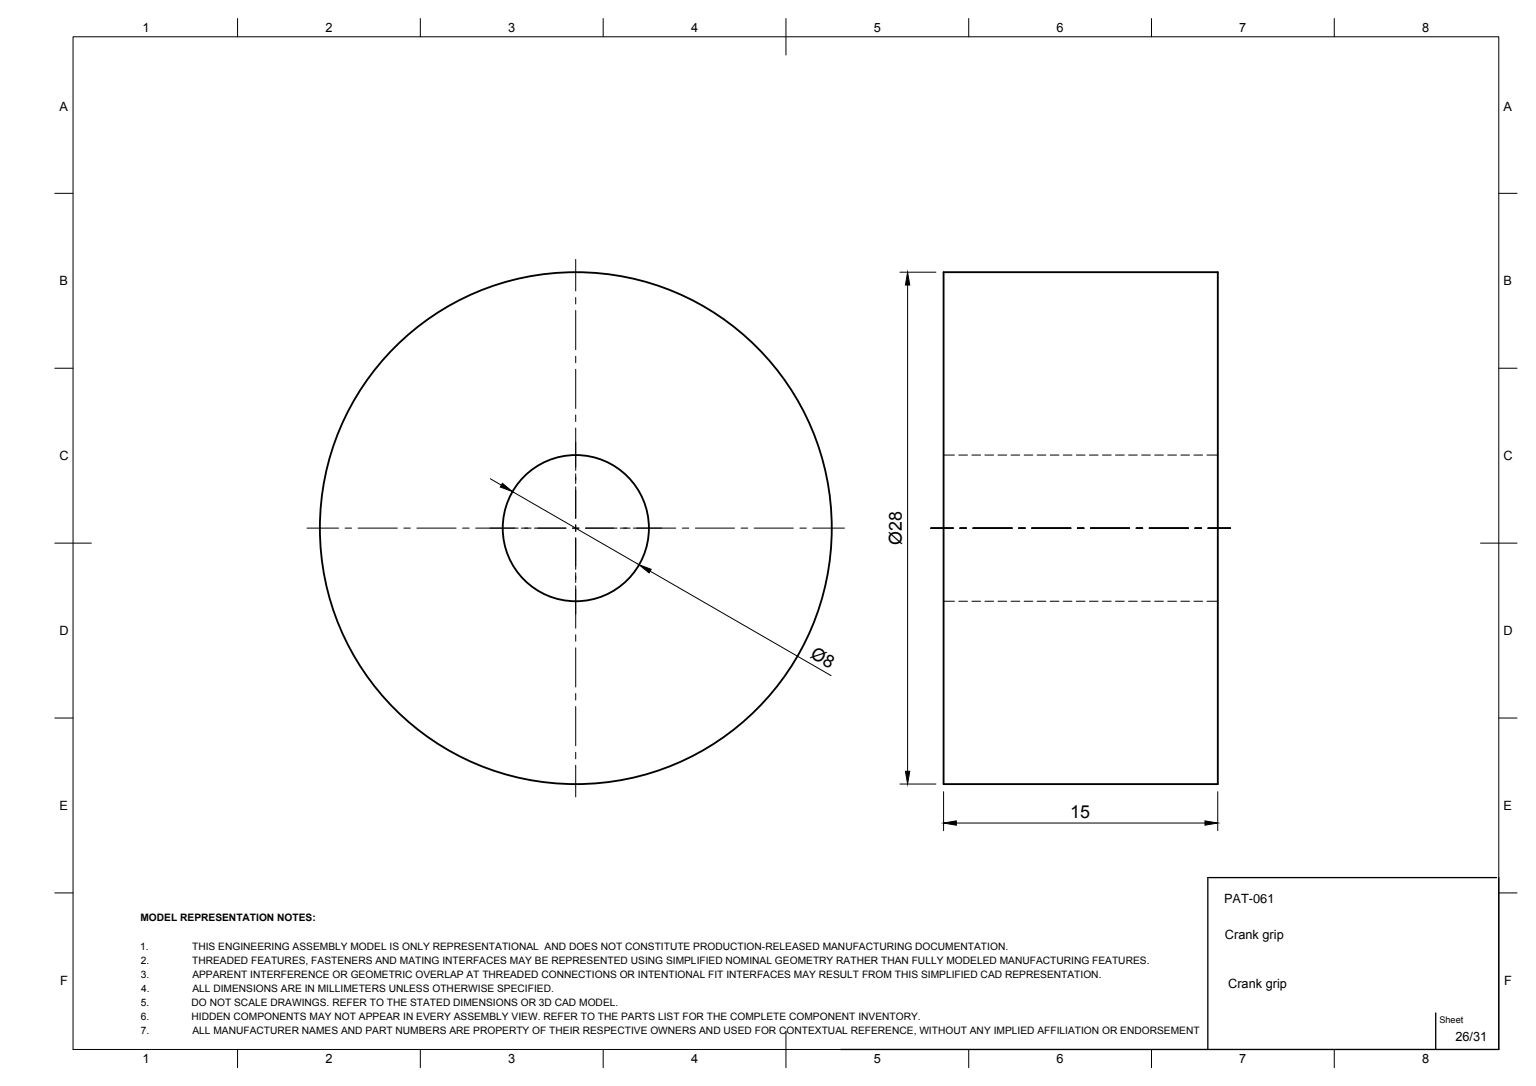
ISO-10303-21;
HEADER;
/* Generated by software containing ST-Developer
 * from STEP Tools, Inc. (www.steptools.com) 
 */

FILE_DESCRIPTION(
/* description */ ('Compact intermittent indexer'),
/* implementation_level */ '2;1');

FILE_NAME(
/* name */ 'Crank grip.step',
/* time_stamp */ '2026-10-29T16:32:17-07:00',
/* author */ (''),
/* organization */ (''),
/* preprocessor_version */ 'ST-DEVELOPER v20.2',
/* originating_system */ 'Autodesk Translation Framework v15.17.0.0',
/* authorisation */ '');

FILE_SCHEMA (('AUTOMOTIVE_DESIGN { 1 0 10303 214 3 1 1 }'));
ENDSEC;

DATA;
#10=MECHANICAL_DESIGN_GEOMETRIC_PRESENTATION_REPRESENTATION('',(#283),#10837);
#227=SHAPE_REPRESENTATION_RELATIONSHIP('SRR','None',#10963,#251);
#251=ADVANCED_BREP_SHAPE_REPRESENTATION('',(#314),#10830);
#283=STYLED_ITEM('',(#11173),#314);
#314=MANIFOLD_SOLID_BREP('Body1',#5656);
#452=FACE_BOUND('',#1314,.T.);
#453=FACE_BOUND('',#1316,.T.);
#587=PLANE('',#6441);
#588=PLANE('',#6442);
#884=FACE_OUTER_BOUND('',#1311,.T.);
#885=FACE_OUTER_BOUND('',#1312,.T.);
#886=FACE_OUTER_BOUND('',#1313,.T.);
#887=FACE_OUTER_BOUND('',#1315,.T.);
#1311=EDGE_LOOP('',(#4660,#4661,#4662,#4663));
#1312=EDGE_LOOP('',(#4664,#4665,#4666,#4667));
#1313=EDGE_LOOP('',(#4668));
#1314=EDGE_LOOP('',(#4669));
#1315=EDGE_LOOP('',(#4670));
#1316=EDGE_LOOP('',(#4671));
#1631=LINE('',#10091,#1989);
#1632=LINE('',#10097,#1990);
#1989=VECTOR('',#7883,0.4);
#1990=VECTOR('',#7890,1.4);
#2395=CIRCLE('',#6436,0.4);
#2396=CIRCLE('',#6437,0.4);
#2397=CIRCLE('',#6439,1.4);
#2398=CIRCLE('',#6440,1.4);
#2807=VERTEX_POINT('',#10088);
#2808=VERTEX_POINT('',#10090);
#2809=VERTEX_POINT('',#10094);
#2810=VERTEX_POINT('',#10096);
#3452=EDGE_CURVE('',#2807,#2807,#2395,.T.);
#3453=EDGE_CURVE('',#2807,#2808,#1631,.T.);
#3454=EDGE_CURVE('',#2808,#2808,#2396,.T.);
#3455=EDGE_CURVE('',#2809,#2809,#2397,.T.);
#3456=EDGE_CURVE('',#2809,#2810,#1632,.T.);
#3457=EDGE_CURVE('',#2810,#2810,#2398,.T.);
#4660=ORIENTED_EDGE('',*,*,#3452,.F.);
#4661=ORIENTED_EDGE('',*,*,#3453,.T.);
#4662=ORIENTED_EDGE('',*,*,#3454,.T.);
#4663=ORIENTED_EDGE('',*,*,#3453,.F.);
#4664=ORIENTED_EDGE('',*,*,#3455,.F.);
#4665=ORIENTED_EDGE('',*,*,#3456,.T.);
#4666=ORIENTED_EDGE('',*,*,#3457,.T.);
#4667=ORIENTED_EDGE('',*,*,#3456,.F.);
#4668=ORIENTED_EDGE('',*,*,#3455,.T.);
#4669=ORIENTED_EDGE('',*,*,#3452,.T.);
#4670=ORIENTED_EDGE('',*,*,#3457,.F.);
#4671=ORIENTED_EDGE('',*,*,#3454,.F.);
#5262=CYLINDRICAL_SURFACE('',#6435,0.4);
#5263=CYLINDRICAL_SURFACE('',#6438,1.4);
#5527=ADVANCED_FACE('',(#884),#5262,.F.);
#5528=ADVANCED_FACE('',(#885),#5263,.T.);
#5529=ADVANCED_FACE('',(#886,#452),#587,.T.);
#5530=ADVANCED_FACE('',(#887,#453),#588,.F.);
#5656=CLOSED_SHELL('',(#5527,#5528,#5529,#5530));
#6434=AXIS2_PLACEMENT_3D('',#10086,#7877,#7878);
#6435=AXIS2_PLACEMENT_3D('',#10087,#7879,#7880);
#6436=AXIS2_PLACEMENT_3D('',#10089,#7881,#7882);
#6437=AXIS2_PLACEMENT_3D('',#10092,#7884,#7885);
#6438=AXIS2_PLACEMENT_3D('',#10093,#7886,#7887);
#6439=AXIS2_PLACEMENT_3D('',#10095,#7888,#7889);
#6440=AXIS2_PLACEMENT_3D('',#10098,#7891,#7892);
#6441=AXIS2_PLACEMENT_3D('',#10099,#7893,#7894);
#6442=AXIS2_PLACEMENT_3D('',#10100,#7895,#7896);
#7877=DIRECTION('axis',(0.,0.,1.));
#7878=DIRECTION('refdir',(1.,0.,0.));
#7879=DIRECTION('center_axis',(0.,0.,1.));
#7880=DIRECTION('ref_axis',(1.,0.,0.));
#7881=DIRECTION('center_axis',(0.,0.,-1.));
#7882=DIRECTION('ref_axis',(1.,0.,0.));
#7883=DIRECTION('',(0.,0.,-1.));
#7884=DIRECTION('center_axis',(0.,0.,-1.));
#7885=DIRECTION('ref_axis',(1.,0.,0.));
#7886=DIRECTION('center_axis',(0.,0.,1.));
#7887=DIRECTION('ref_axis',(1.,0.,0.));
#7888=DIRECTION('center_axis',(0.,0.,1.));
#7889=DIRECTION('ref_axis',(1.,0.,0.));
#7890=DIRECTION('',(0.,0.,-1.));
#7891=DIRECTION('center_axis',(0.,0.,1.));
#7892=DIRECTION('ref_axis',(1.,0.,0.));
#7893=DIRECTION('center_axis',(0.,0.,1.));
#7894=DIRECTION('ref_axis',(1.,0.,0.));
#7895=DIRECTION('center_axis',(0.,0.,1.));
#7896=DIRECTION('ref_axis',(1.,0.,0.));
#10086=CARTESIAN_POINT('',(0.,0.,0.));
#10087=CARTESIAN_POINT('Origin',(0.,0.,7.));
#10088=CARTESIAN_POINT('',(-0.4,-4.89858719658941E-17,8.5));
#10089=CARTESIAN_POINT('Origin',(0.,0.,8.5));
#10090=CARTESIAN_POINT('',(-0.4,-4.89858719658941E-17,7.));
#10091=CARTESIAN_POINT('',(-0.4,-4.89858719658941E-17,7.));
#10092=CARTESIAN_POINT('Origin',(0.,0.,7.));
#10093=CARTESIAN_POINT('Origin',(0.,0.,7.));
#10094=CARTESIAN_POINT('',(-1.4,-1.71450551880629E-16,8.5));
#10095=CARTESIAN_POINT('Origin',(0.,0.,8.5));
#10096=CARTESIAN_POINT('',(-1.4,-1.71450551880629E-16,7.));
#10097=CARTESIAN_POINT('',(-1.4,-1.71450551880629E-16,7.));
#10098=CARTESIAN_POINT('Origin',(0.,0.,7.));
#10099=CARTESIAN_POINT('Origin',(0.,0.,8.5));
#10100=CARTESIAN_POINT('Origin',(0.,0.,7.));
#10800=UNCERTAINTY_MEASURE_WITH_UNIT(LENGTH_MEASURE(0.001),#10838,
'DISTANCE_ACCURACY_VALUE',
'Maximum model space distance between geometric entities at asserted c
onnectivities');
#10807=UNCERTAINTY_MEASURE_WITH_UNIT(LENGTH_MEASURE(0.001),#10838,
'DISTANCE_ACCURACY_VALUE',
'Maximum model space distance between geometric entities at asserted c
onnectivities');
#10830=(
GEOMETRIC_REPRESENTATION_CONTEXT(3)
GLOBAL_UNCERTAINTY_ASSIGNED_CONTEXT((#10800))
GLOBAL_UNIT_ASSIGNED_CONTEXT((#10838,#10840,#10841))
REPRESENTATION_CONTEXT('','3D')
);
#10837=(
GEOMETRIC_REPRESENTATION_CONTEXT(3)
GLOBAL_UNCERTAINTY_ASSIGNED_CONTEXT((#10807))
GLOBAL_UNIT_ASSIGNED_CONTEXT((#10838,#10840,#10841))
REPRESENTATION_CONTEXT('','3D')
);
#10838=(
LENGTH_UNIT()
NAMED_UNIT(*)
SI_UNIT(.CENTI.,.METRE.)
);
#10840=(
NAMED_UNIT(*)
PLANE_ANGLE_UNIT()
SI_UNIT($,.RADIAN.)
);
#10841=(
NAMED_UNIT(*)
SI_UNIT($,.STERADIAN.)
SOLID_ANGLE_UNIT()
);
#10864=SHAPE_DEFINITION_REPRESENTATION(#10898,#10963);
#10898=PRODUCT_DEFINITION_SHAPE('',$,#10993);
#10963=SHAPE_REPRESENTATION('',(#6434),#10830);
#10970=PRODUCT_DEFINITION_CONTEXT('part definition',#11059,'design');
#10993=PRODUCT_DEFINITION('Crank grip','Crank grip',#11022,#10970);
#11022=PRODUCT_DEFINITION_FORMATION('',$,#11083);
#11059=APPLICATION_CONTEXT(
'Core Data for Automotive Mechanical Design Process');
#11060=PRODUCT_CONTEXT('part definition',#11059,'mechanical');
#11083=PRODUCT('Crank grip','Crank grip','Crank grip',(#11060));
#11167=COLOUR_RGB('Black',0.12,0.14,0.17);
#11168=FILL_AREA_STYLE_COLOUR('',#11167);
#11169=FILL_AREA_STYLE('',(#11168));
#11170=SURFACE_STYLE_FILL_AREA(#11169);
#11171=SURFACE_SIDE_STYLE('',(#11170));
#11172=SURFACE_STYLE_USAGE(.BOTH.,#11171);
#11173=PRESENTATION_STYLE_ASSIGNMENT((#11172));
ENDSEC;
END-ISO-10303-21;
